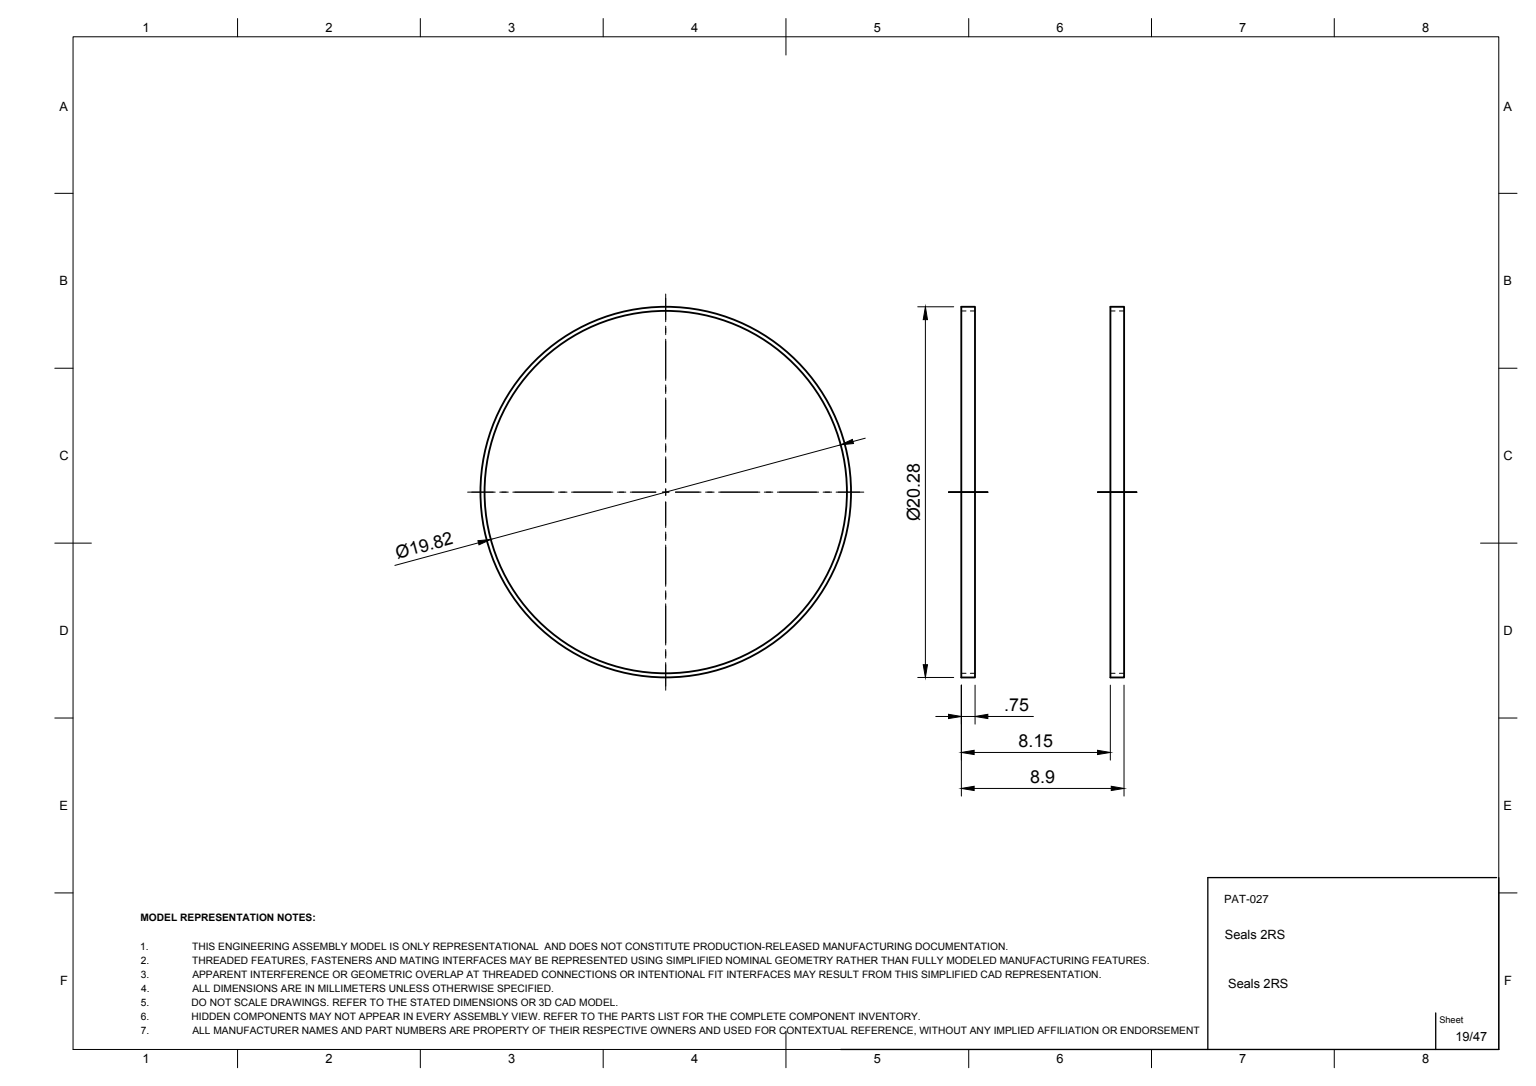
ISO-10303-21;
HEADER;
/* Generated by software containing ST-Developer
 * from STEP Tools, Inc. (www.steptools.com) 
 */

FILE_DESCRIPTION(
/* description */ ('Crank-driven oscillating fan base (mechanism only)'),

/* implementation_level */ '2;1');

FILE_NAME(
/* name */ 'Seals 2RS.step',
/* time_stamp */ '2026-10-28T03:25:00-07:00',
/* author */ (''),
/* organization */ (''),
/* preprocessor_version */ 'ST-DEVELOPER v20.2',
/* originating_system */ 'Autodesk Translation Framework v15.17.0.0',
/* authorisation */ '');

FILE_SCHEMA (('AUTOMOTIVE_DESIGN { 1 0 10303 214 3 1 1 }'));
ENDSEC;

DATA;
#10=MECHANICAL_DESIGN_GEOMETRIC_PRESENTATION_REPRESENTATION('',(#457,#458),#11916);
#370=SHAPE_REPRESENTATION_RELATIONSHIP('SRR','None',#12095,#410);
#410=ADVANCED_BREP_SHAPE_REPRESENTATION('',(#504,#505),#11886);
#457=STYLED_ITEM('',(#12375),#504);
#458=STYLED_ITEM('',(#12375),#505);
#504=MANIFOLD_SOLID_BREP('Body1',#6088);
#505=MANIFOLD_SOLID_BREP('Body2',#6089);
#612=FACE_BOUND('',#1511,.T.);
#613=FACE_BOUND('',#1514,.T.);
#614=FACE_BOUND('',#1517,.T.);
#615=FACE_BOUND('',#1520,.T.);
#766=PLANE('',#6942);
#767=PLANE('',#6947);
#768=PLANE('',#6950);
#769=PLANE('',#6955);
#1053=FACE_OUTER_BOUND('',#1510,.T.);
#1054=FACE_OUTER_BOUND('',#1512,.T.);
#1055=FACE_OUTER_BOUND('',#1513,.T.);
#1056=FACE_OUTER_BOUND('',#1515,.T.);
#1057=FACE_OUTER_BOUND('',#1516,.T.);
#1058=FACE_OUTER_BOUND('',#1518,.T.);
#1059=FACE_OUTER_BOUND('',#1519,.T.);
#1060=FACE_OUTER_BOUND('',#1521,.T.);
#1510=EDGE_LOOP('',(#4792));
#1511=EDGE_LOOP('',(#4793));
#1512=EDGE_LOOP('',(#4794,#4795,#4796,#4797));
#1513=EDGE_LOOP('',(#4798));
#1514=EDGE_LOOP('',(#4799));
#1515=EDGE_LOOP('',(#4800,#4801,#4802,#4803));
#1516=EDGE_LOOP('',(#4804));
#1517=EDGE_LOOP('',(#4805));
#1518=EDGE_LOOP('',(#4806,#4807,#4808,#4809));
#1519=EDGE_LOOP('',(#4810));
#1520=EDGE_LOOP('',(#4811));
#1521=EDGE_LOOP('',(#4812,#4813,#4814,#4815));
#1935=LINE('',#10727,#2268);
#1936=LINE('',#10732,#2269);
#1937=LINE('',#10741,#2270);
#1938=LINE('',#10746,#2271);
#2268=VECTOR('',#8324,1.013815);
#2269=VECTOR('',#8331,0.991185);
#2270=VECTOR('',#8342,1.013815);
#2271=VECTOR('',#8349,0.991185);
#2663=CIRCLE('',#6943,1.013815);
#2664=CIRCLE('',#6944,0.991185);
#2665=CIRCLE('',#6946,1.013815);
#2666=CIRCLE('',#6948,0.991185);
#2667=CIRCLE('',#6951,1.013815);
#2668=CIRCLE('',#6952,0.991185);
#2669=CIRCLE('',#6954,1.013815);
#2670=CIRCLE('',#6956,0.991185);
#3080=VERTEX_POINT('',#10720);
#3081=VERTEX_POINT('',#10722);
#3082=VERTEX_POINT('',#10725);
#3083=VERTEX_POINT('',#10729);
#3084=VERTEX_POINT('',#10734);
#3085=VERTEX_POINT('',#10736);
#3086=VERTEX_POINT('',#10739);
#3087=VERTEX_POINT('',#10743);
#3691=EDGE_CURVE('',#3080,#3080,#2663,.T.);
#3692=EDGE_CURVE('',#3081,#3081,#2664,.T.);
#3693=EDGE_CURVE('',#3082,#3082,#2665,.T.);
#3694=EDGE_CURVE('',#3082,#3080,#1935,.T.);
#3695=EDGE_CURVE('',#3083,#3083,#2666,.T.);
#3696=EDGE_CURVE('',#3083,#3081,#1936,.T.);
#3697=EDGE_CURVE('',#3084,#3084,#2667,.T.);
#3698=EDGE_CURVE('',#3085,#3085,#2668,.T.);
#3699=EDGE_CURVE('',#3086,#3086,#2669,.T.);
#3700=EDGE_CURVE('',#3086,#3084,#1937,.T.);
#3701=EDGE_CURVE('',#3087,#3087,#2670,.T.);
#3702=EDGE_CURVE('',#3087,#3085,#1938,.T.);
#4792=ORIENTED_EDGE('',*,*,#3691,.F.);
#4793=ORIENTED_EDGE('',*,*,#3692,.T.);
#4794=ORIENTED_EDGE('',*,*,#3693,.F.);
#4795=ORIENTED_EDGE('',*,*,#3694,.T.);
#4796=ORIENTED_EDGE('',*,*,#3691,.T.);
#4797=ORIENTED_EDGE('',*,*,#3694,.F.);
#4798=ORIENTED_EDGE('',*,*,#3693,.T.);
#4799=ORIENTED_EDGE('',*,*,#3695,.F.);
#4800=ORIENTED_EDGE('',*,*,#3695,.T.);
#4801=ORIENTED_EDGE('',*,*,#3696,.T.);
#4802=ORIENTED_EDGE('',*,*,#3692,.F.);
#4803=ORIENTED_EDGE('',*,*,#3696,.F.);
#4804=ORIENTED_EDGE('',*,*,#3697,.F.);
#4805=ORIENTED_EDGE('',*,*,#3698,.T.);
#4806=ORIENTED_EDGE('',*,*,#3699,.F.);
#4807=ORIENTED_EDGE('',*,*,#3700,.T.);
#4808=ORIENTED_EDGE('',*,*,#3697,.T.);
#4809=ORIENTED_EDGE('',*,*,#3700,.F.);
#4810=ORIENTED_EDGE('',*,*,#3699,.T.);
#4811=ORIENTED_EDGE('',*,*,#3701,.F.);
#4812=ORIENTED_EDGE('',*,*,#3701,.T.);
#4813=ORIENTED_EDGE('',*,*,#3702,.T.);
#4814=ORIENTED_EDGE('',*,*,#3698,.F.);
#4815=ORIENTED_EDGE('',*,*,#3702,.F.);
#5614=CYLINDRICAL_SURFACE('',#6945,1.013815);
#5615=CYLINDRICAL_SURFACE('',#6949,0.991185);
#5616=CYLINDRICAL_SURFACE('',#6953,1.013815);
#5617=CYLINDRICAL_SURFACE('',#6957,0.991185);
#5859=ADVANCED_FACE('',(#1053,#612),#766,.T.);
#5860=ADVANCED_FACE('',(#1054),#5614,.T.);
#5861=ADVANCED_FACE('',(#1055,#613),#767,.T.);
#5862=ADVANCED_FACE('',(#1056),#5615,.F.);
#5863=ADVANCED_FACE('',(#1057,#614),#768,.T.);
#5864=ADVANCED_FACE('',(#1058),#5616,.T.);
#5865=ADVANCED_FACE('',(#1059,#615),#769,.T.);
#5866=ADVANCED_FACE('',(#1060),#5617,.F.);
#6088=CLOSED_SHELL('',(#5859,#5860,#5861,#5862));
#6089=CLOSED_SHELL('',(#5863,#5864,#5865,#5866));
#6941=AXIS2_PLACEMENT_3D('',#10718,#8312,#8313);
#6942=AXIS2_PLACEMENT_3D('',#10719,#8314,#8315);
#6943=AXIS2_PLACEMENT_3D('',#10721,#8316,#8317);
#6944=AXIS2_PLACEMENT_3D('',#10723,#8318,#8319);
#6945=AXIS2_PLACEMENT_3D('',#10724,#8320,#8321);
#6946=AXIS2_PLACEMENT_3D('',#10726,#8322,#8323);
#6947=AXIS2_PLACEMENT_3D('',#10728,#8325,#8326);
#6948=AXIS2_PLACEMENT_3D('',#10730,#8327,#8328);
#6949=AXIS2_PLACEMENT_3D('',#10731,#8329,#8330);
#6950=AXIS2_PLACEMENT_3D('',#10733,#8332,#8333);
#6951=AXIS2_PLACEMENT_3D('',#10735,#8334,#8335);
#6952=AXIS2_PLACEMENT_3D('',#10737,#8336,#8337);
#6953=AXIS2_PLACEMENT_3D('',#10738,#8338,#8339);
#6954=AXIS2_PLACEMENT_3D('',#10740,#8340,#8341);
#6955=AXIS2_PLACEMENT_3D('',#10742,#8343,#8344);
#6956=AXIS2_PLACEMENT_3D('',#10744,#8345,#8346);
#6957=AXIS2_PLACEMENT_3D('',#10745,#8347,#8348);
#8312=DIRECTION('axis',(0.,0.,1.));
#8313=DIRECTION('refdir',(1.,0.,0.));
#8314=DIRECTION('center_axis',(0.,1.,0.));
#8315=DIRECTION('ref_axis',(0.,0.,1.));
#8316=DIRECTION('center_axis',(0.,-1.,0.));
#8317=DIRECTION('ref_axis',(1.,0.,0.));
#8318=DIRECTION('center_axis',(0.,-1.,0.));
#8319=DIRECTION('ref_axis',(1.,0.,0.));
#8320=DIRECTION('center_axis',(0.,-1.,0.));
#8321=DIRECTION('ref_axis',(1.,0.,0.));
#8322=DIRECTION('center_axis',(0.,-1.,0.));
#8323=DIRECTION('ref_axis',(1.,0.,0.));
#8324=DIRECTION('',(0.,1.,0.));
#8325=DIRECTION('center_axis',(0.,-1.,0.));
#8326=DIRECTION('ref_axis',(0.,0.,-1.));
#8327=DIRECTION('center_axis',(0.,-1.,0.));
#8328=DIRECTION('ref_axis',(1.,0.,0.));
#8329=DIRECTION('center_axis',(0.,-1.,0.));
#8330=DIRECTION('ref_axis',(1.,0.,0.));
#8331=DIRECTION('',(0.,1.,0.));
#8332=DIRECTION('center_axis',(0.,1.,0.));
#8333=DIRECTION('ref_axis',(0.,0.,1.));
#8334=DIRECTION('center_axis',(0.,-1.,0.));
#8335=DIRECTION('ref_axis',(1.,0.,0.));
#8336=DIRECTION('center_axis',(0.,-1.,0.));
#8337=DIRECTION('ref_axis',(1.,0.,0.));
#8338=DIRECTION('center_axis',(0.,-1.,0.));
#8339=DIRECTION('ref_axis',(1.,0.,0.));
#8340=DIRECTION('center_axis',(0.,-1.,0.));
#8341=DIRECTION('ref_axis',(1.,0.,0.));
#8342=DIRECTION('',(0.,1.,0.));
#8343=DIRECTION('center_axis',(0.,-1.,0.));
#8344=DIRECTION('ref_axis',(0.,0.,-1.));
#8345=DIRECTION('center_axis',(0.,-1.,0.));
#8346=DIRECTION('ref_axis',(1.,0.,0.));
#8347=DIRECTION('center_axis',(0.,-1.,0.));
#8348=DIRECTION('ref_axis',(1.,0.,0.));
#8349=DIRECTION('',(0.,1.,0.));
#10718=CARTESIAN_POINT('',(0.,0.,0.));
#10719=CARTESIAN_POINT('Origin',(1.013815,0.445,0.));
#10720=CARTESIAN_POINT('',(-1.013815,0.445,-1.24156529467757E-16));
#10721=CARTESIAN_POINT('Origin',(0.,0.445,0.));
#10722=CARTESIAN_POINT('',(-0.991185,0.445,-1.21385153761287E-16));
#10723=CARTESIAN_POINT('Origin',(0.,0.445,0.));
#10724=CARTESIAN_POINT('Origin',(0.,0.4075,0.));
#10725=CARTESIAN_POINT('',(-1.013815,0.37,-1.24156529467757E-16));
#10726=CARTESIAN_POINT('Origin',(0.,0.37,0.));
#10727=CARTESIAN_POINT('',(-1.013815,0.4075,-1.24156529467757E-16));
#10728=CARTESIAN_POINT('Origin',(0.991185,0.37,0.));
#10729=CARTESIAN_POINT('',(-0.991185,0.37,-1.21385153761287E-16));
#10730=CARTESIAN_POINT('Origin',(0.,0.37,0.));
#10731=CARTESIAN_POINT('Origin',(0.,0.4075,0.));
#10732=CARTESIAN_POINT('',(-0.991185,0.4075,-1.21385153761287E-16));
#10733=CARTESIAN_POINT('Origin',(1.013815,-0.37,0.));
#10734=CARTESIAN_POINT('',(-1.013815,-0.37,-1.24156529467757E-16));
#10735=CARTESIAN_POINT('Origin',(0.,-0.37,0.));
#10736=CARTESIAN_POINT('',(-0.991185,-0.37,-1.21385153761287E-16));
#10737=CARTESIAN_POINT('Origin',(0.,-0.37,0.));
#10738=CARTESIAN_POINT('Origin',(0.,-0.4075,0.));
#10739=CARTESIAN_POINT('',(-1.013815,-0.445,-1.24156529467757E-16));
#10740=CARTESIAN_POINT('Origin',(0.,-0.445,0.));
#10741=CARTESIAN_POINT('',(-1.013815,-0.4075,-1.24156529467757E-16));
#10742=CARTESIAN_POINT('Origin',(0.991185,-0.445,0.));
#10743=CARTESIAN_POINT('',(-0.991185,-0.445,-1.21385153761287E-16));
#10744=CARTESIAN_POINT('Origin',(0.,-0.445,0.));
#10745=CARTESIAN_POINT('Origin',(0.,-0.4075,0.));
#10746=CARTESIAN_POINT('',(-0.991185,-0.4075,-1.21385153761287E-16));
#11839=UNCERTAINTY_MEASURE_WITH_UNIT(LENGTH_MEASURE(0.001),#11917,
'DISTANCE_ACCURACY_VALUE',
'Maximum model space distance between geometric entities at asserted c
onnectivities');
#11869=UNCERTAINTY_MEASURE_WITH_UNIT(LENGTH_MEASURE(0.001),#11917,
'DISTANCE_ACCURACY_VALUE',
'Maximum model space distance between geometric entities at asserted c
onnectivities');
#11886=(
GEOMETRIC_REPRESENTATION_CONTEXT(3)
GLOBAL_UNCERTAINTY_ASSIGNED_CONTEXT((#11839))
GLOBAL_UNIT_ASSIGNED_CONTEXT((#11917,#11919,#11920))
REPRESENTATION_CONTEXT('','3D')
);
#11916=(
GEOMETRIC_REPRESENTATION_CONTEXT(3)
GLOBAL_UNCERTAINTY_ASSIGNED_CONTEXT((#11869))
GLOBAL_UNIT_ASSIGNED_CONTEXT((#11917,#11919,#11920))
REPRESENTATION_CONTEXT('','3D')
);
#11917=(
LENGTH_UNIT()
NAMED_UNIT(*)
SI_UNIT(.CENTI.,.METRE.)
);
#11919=(
NAMED_UNIT(*)
PLANE_ANGLE_UNIT()
SI_UNIT($,.RADIAN.)
);
#11920=(
NAMED_UNIT(*)
SI_UNIT($,.STERADIAN.)
SOLID_ANGLE_UNIT()
);
#11937=SHAPE_DEFINITION_REPRESENTATION(#11983,#12095);
#11983=PRODUCT_DEFINITION_SHAPE('',$,#12142);
#12095=SHAPE_REPRESENTATION('',(#6941),#11886);
#12125=PRODUCT_DEFINITION_CONTEXT('part definition',#12265,'design');
#12142=PRODUCT_DEFINITION('Seals 2RS','Seals 2RS',#12188,#12125);
#12188=PRODUCT_DEFINITION_FORMATION('',$,#12283);
#12265=APPLICATION_CONTEXT(
'Core Data for Automotive Mechanical Design Process');
#12266=PRODUCT_CONTEXT('part definition',#12265,'mechanical');
#12283=PRODUCT('Seals 2RS','Seals 2RS','Seals 2RS',(#12266));
#12369=COLOUR_RGB('Grey',0.48,0.52,0.57);
#12370=FILL_AREA_STYLE_COLOUR('',#12369);
#12371=FILL_AREA_STYLE('',(#12370));
#12372=SURFACE_STYLE_FILL_AREA(#12371);
#12373=SURFACE_SIDE_STYLE('',(#12372));
#12374=SURFACE_STYLE_USAGE(.BOTH.,#12373);
#12375=PRESENTATION_STYLE_ASSIGNMENT((#12374));
ENDSEC;
END-ISO-10303-21;
